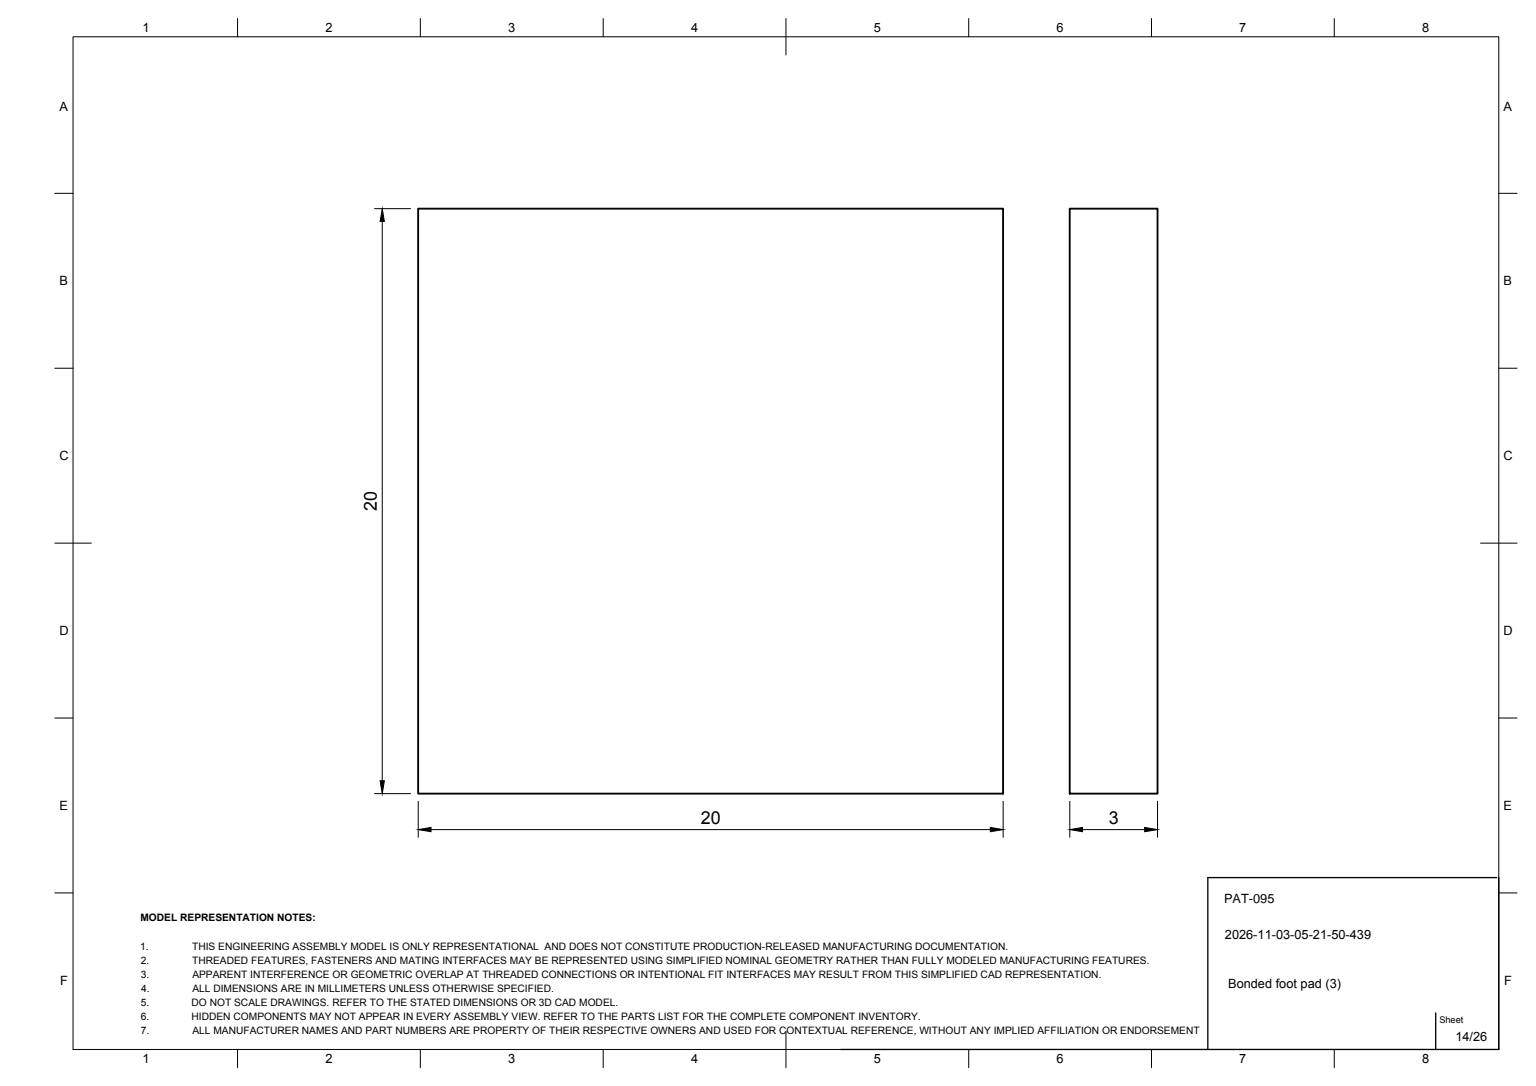
ISO-10303-21;
HEADER;
/* Generated by software containing ST-Developer
 * from STEP Tools, Inc. (www.steptools.com) 
 */

FILE_DESCRIPTION(
/* description */ ('Single-Axis Profile-Rail Linear Slide'),
/* implementation_level */ '2;1');

FILE_NAME(
/* name */ 'Bonded foot pad (3).step',
/* time_stamp */ '2026-10-27T10:47:43-07:00',
/* author */ (''),
/* organization */ (''),
/* preprocessor_version */ 'ST-DEVELOPER v20.2',
/* originating_system */ 'Autodesk Translation Framework v15.17.0.0',
/* authorisation */ '');

FILE_SCHEMA (('AUTOMOTIVE_DESIGN { 1 0 10303 214 3 1 1 }'));
ENDSEC;

DATA;
#10=MECHANICAL_DESIGN_GEOMETRIC_PRESENTATION_REPRESENTATION('',(#338),#14478);
#284=SHAPE_REPRESENTATION_RELATIONSHIP('SRR','None',#14614,#311);
#311=ADVANCED_BREP_SHAPE_REPRESENTATION('',(#365),#14458);
#338=STYLED_ITEM('',(#14824),#365);
#365=MANIFOLD_SOLID_BREP('Body1',#8598);
#642=PLANE('',#9177);
#643=PLANE('',#9178);
#644=PLANE('',#9179);
#645=PLANE('',#9180);
#646=PLANE('',#9181);
#647=PLANE('',#9182);
#1038=FACE_OUTER_BOUND('',#1537,.T.);
#1039=FACE_OUTER_BOUND('',#1538,.T.);
#1040=FACE_OUTER_BOUND('',#1539,.T.);
#1041=FACE_OUTER_BOUND('',#1540,.T.);
#1042=FACE_OUTER_BOUND('',#1541,.T.);
#1043=FACE_OUTER_BOUND('',#1542,.T.);
#1537=EDGE_LOOP('',(#6869,#6870,#6871,#6872));
#1538=EDGE_LOOP('',(#6873,#6874,#6875,#6876));
#1539=EDGE_LOOP('',(#6877,#6878,#6879,#6880));
#1540=EDGE_LOOP('',(#6881,#6882,#6883,#6884));
#1541=EDGE_LOOP('',(#6885,#6886,#6887,#6888));
#1542=EDGE_LOOP('',(#6889,#6890,#6891,#6892));
#2320=LINE('',#13089,#3291);
#2321=LINE('',#13091,#3292);
#2322=LINE('',#13093,#3293);
#2323=LINE('',#13094,#3294);
#2324=LINE('',#13097,#3295);
#2325=LINE('',#13099,#3296);
#2326=LINE('',#13100,#3297);
#2327=LINE('',#13103,#3298);
#2328=LINE('',#13105,#3299);
#2329=LINE('',#13106,#3300);
#2330=LINE('',#13108,#3301);
#2331=LINE('',#13109,#3302);
#3291=VECTOR('',#10619,1.);
#3292=VECTOR('',#10620,1.);
#3293=VECTOR('',#10621,1.);
#3294=VECTOR('',#10622,1.);
#3295=VECTOR('',#10625,1.);
#3296=VECTOR('',#10626,1.);
#3297=VECTOR('',#10627,1.);
#3298=VECTOR('',#10630,1.);
#3299=VECTOR('',#10631,1.);
#3300=VECTOR('',#10632,1.);
#3301=VECTOR('',#10635,1.);
#3302=VECTOR('',#10636,1.);
#4290=VERTEX_POINT('',#13087);
#4291=VERTEX_POINT('',#13088);
#4292=VERTEX_POINT('',#13090);
#4293=VERTEX_POINT('',#13092);
#4294=VERTEX_POINT('',#13096);
#4295=VERTEX_POINT('',#13098);
#4296=VERTEX_POINT('',#13102);
#4297=VERTEX_POINT('',#13104);
#5212=EDGE_CURVE('',#4290,#4291,#2320,.T.);
#5213=EDGE_CURVE('',#4291,#4292,#2321,.T.);
#5214=EDGE_CURVE('',#4293,#4292,#2322,.T.);
#5215=EDGE_CURVE('',#4290,#4293,#2323,.T.);
#5216=EDGE_CURVE('',#4294,#4290,#2324,.T.);
#5217=EDGE_CURVE('',#4295,#4293,#2325,.T.);
#5218=EDGE_CURVE('',#4294,#4295,#2326,.T.);
#5219=EDGE_CURVE('',#4296,#4294,#2327,.T.);
#5220=EDGE_CURVE('',#4297,#4295,#2328,.T.);
#5221=EDGE_CURVE('',#4296,#4297,#2329,.T.);
#5222=EDGE_CURVE('',#4291,#4296,#2330,.T.);
#5223=EDGE_CURVE('',#4292,#4297,#2331,.T.);
#6869=ORIENTED_EDGE('',*,*,#5212,.T.);
#6870=ORIENTED_EDGE('',*,*,#5213,.T.);
#6871=ORIENTED_EDGE('',*,*,#5214,.F.);
#6872=ORIENTED_EDGE('',*,*,#5215,.F.);
#6873=ORIENTED_EDGE('',*,*,#5216,.T.);
#6874=ORIENTED_EDGE('',*,*,#5215,.T.);
#6875=ORIENTED_EDGE('',*,*,#5217,.F.);
#6876=ORIENTED_EDGE('',*,*,#5218,.F.);
#6877=ORIENTED_EDGE('',*,*,#5219,.T.);
#6878=ORIENTED_EDGE('',*,*,#5218,.T.);
#6879=ORIENTED_EDGE('',*,*,#5220,.F.);
#6880=ORIENTED_EDGE('',*,*,#5221,.F.);
#6881=ORIENTED_EDGE('',*,*,#5222,.T.);
#6882=ORIENTED_EDGE('',*,*,#5221,.T.);
#6883=ORIENTED_EDGE('',*,*,#5223,.F.);
#6884=ORIENTED_EDGE('',*,*,#5213,.F.);
#6885=ORIENTED_EDGE('',*,*,#5223,.T.);
#6886=ORIENTED_EDGE('',*,*,#5220,.T.);
#6887=ORIENTED_EDGE('',*,*,#5217,.T.);
#6888=ORIENTED_EDGE('',*,*,#5214,.T.);
#6889=ORIENTED_EDGE('',*,*,#5222,.F.);
#6890=ORIENTED_EDGE('',*,*,#5212,.F.);
#6891=ORIENTED_EDGE('',*,*,#5216,.F.);
#6892=ORIENTED_EDGE('',*,*,#5219,.F.);
#8332=ADVANCED_FACE('',(#1038),#642,.T.);
#8333=ADVANCED_FACE('',(#1039),#643,.T.);
#8334=ADVANCED_FACE('',(#1040),#644,.T.);
#8335=ADVANCED_FACE('',(#1041),#645,.T.);
#8336=ADVANCED_FACE('',(#1042),#646,.T.);
#8337=ADVANCED_FACE('',(#1043),#647,.F.);
#8598=CLOSED_SHELL('',(#8332,#8333,#8334,#8335,#8336,#8337));
#9176=AXIS2_PLACEMENT_3D('',#13085,#10615,#10616);
#9177=AXIS2_PLACEMENT_3D('',#13086,#10617,#10618);
#9178=AXIS2_PLACEMENT_3D('',#13095,#10623,#10624);
#9179=AXIS2_PLACEMENT_3D('',#13101,#10628,#10629);
#9180=AXIS2_PLACEMENT_3D('',#13107,#10633,#10634);
#9181=AXIS2_PLACEMENT_3D('',#13110,#10637,#10638);
#9182=AXIS2_PLACEMENT_3D('',#13111,#10639,#10640);
#10615=DIRECTION('axis',(0.,0.,1.));
#10616=DIRECTION('refdir',(1.,0.,0.));
#10617=DIRECTION('center_axis',(0.,1.,0.));
#10618=DIRECTION('ref_axis',(-1.,0.,0.));
#10619=DIRECTION('',(-1.,0.,0.));
#10620=DIRECTION('',(0.,0.,1.));
#10621=DIRECTION('',(-1.,0.,0.));
#10622=DIRECTION('',(0.,0.,1.));
#10623=DIRECTION('center_axis',(1.,0.,0.));
#10624=DIRECTION('ref_axis',(0.,1.,0.));
#10625=DIRECTION('',(0.,1.,0.));
#10626=DIRECTION('',(0.,1.,0.));
#10627=DIRECTION('',(0.,0.,1.));
#10628=DIRECTION('center_axis',(0.,-1.,0.));
#10629=DIRECTION('ref_axis',(1.,0.,0.));
#10630=DIRECTION('',(1.,0.,0.));
#10631=DIRECTION('',(1.,0.,0.));
#10632=DIRECTION('',(0.,0.,1.));
#10633=DIRECTION('center_axis',(-1.,0.,0.));
#10634=DIRECTION('ref_axis',(0.,-1.,0.));
#10635=DIRECTION('',(0.,-1.,0.));
#10636=DIRECTION('',(0.,-1.,0.));
#10637=DIRECTION('center_axis',(0.,0.,1.));
#10638=DIRECTION('ref_axis',(1.,0.,0.));
#10639=DIRECTION('center_axis',(0.,0.,1.));
#10640=DIRECTION('ref_axis',(1.,0.,0.));
#13085=CARTESIAN_POINT('',(0.,0.,0.));
#13086=CARTESIAN_POINT('Origin',(20.,4.5,-0.3));
#13087=CARTESIAN_POINT('',(20.,4.5,-0.3));
#13088=CARTESIAN_POINT('',(18.,4.5,-0.3));
#13089=CARTESIAN_POINT('',(20.,4.5,-0.3));
#13090=CARTESIAN_POINT('',(18.,4.5,0.));
#13091=CARTESIAN_POINT('',(18.,4.5,-0.3));
#13092=CARTESIAN_POINT('',(20.,4.5,0.));
#13093=CARTESIAN_POINT('',(20.,4.5,0.));
#13094=CARTESIAN_POINT('',(20.,4.5,-0.3));
#13095=CARTESIAN_POINT('Origin',(20.,2.5,-0.3));
#13096=CARTESIAN_POINT('',(20.,2.5,-0.3));
#13097=CARTESIAN_POINT('',(20.,2.5,-0.3));
#13098=CARTESIAN_POINT('',(20.,2.5,0.));
#13099=CARTESIAN_POINT('',(20.,2.5,0.));
#13100=CARTESIAN_POINT('',(20.,2.5,-0.3));
#13101=CARTESIAN_POINT('Origin',(18.,2.5,-0.3));
#13102=CARTESIAN_POINT('',(18.,2.5,-0.3));
#13103=CARTESIAN_POINT('',(18.,2.5,-0.3));
#13104=CARTESIAN_POINT('',(18.,2.5,0.));
#13105=CARTESIAN_POINT('',(18.,2.5,0.));
#13106=CARTESIAN_POINT('',(18.,2.5,-0.3));
#13107=CARTESIAN_POINT('Origin',(18.,4.5,-0.3));
#13108=CARTESIAN_POINT('',(18.,4.5,-0.3));
#13109=CARTESIAN_POINT('',(18.,4.5,0.));
#13110=CARTESIAN_POINT('Origin',(19.,3.5,0.));
#13111=CARTESIAN_POINT('Origin',(19.,3.5,-0.3));
#14426=UNCERTAINTY_MEASURE_WITH_UNIT(LENGTH_MEASURE(0.001),#14479,
'DISTANCE_ACCURACY_VALUE',
'Maximum model space distance between geometric entities at asserted c
onnectivities');
#14446=UNCERTAINTY_MEASURE_WITH_UNIT(LENGTH_MEASURE(0.001),#14479,
'DISTANCE_ACCURACY_VALUE',
'Maximum model space distance between geometric entities at asserted c
onnectivities');
#14458=(
GEOMETRIC_REPRESENTATION_CONTEXT(3)
GLOBAL_UNCERTAINTY_ASSIGNED_CONTEXT((#14426))
GLOBAL_UNIT_ASSIGNED_CONTEXT((#14479,#14481,#14482))
REPRESENTATION_CONTEXT('','3D')
);
#14478=(
GEOMETRIC_REPRESENTATION_CONTEXT(3)
GLOBAL_UNCERTAINTY_ASSIGNED_CONTEXT((#14446))
GLOBAL_UNIT_ASSIGNED_CONTEXT((#14479,#14481,#14482))
REPRESENTATION_CONTEXT('','3D')
);
#14479=(
LENGTH_UNIT()
NAMED_UNIT(*)
SI_UNIT(.CENTI.,.METRE.)
);
#14481=(
NAMED_UNIT(*)
PLANE_ANGLE_UNIT()
SI_UNIT($,.RADIAN.)
);
#14482=(
NAMED_UNIT(*)
SI_UNIT($,.STERADIAN.)
SOLID_ANGLE_UNIT()
);
#14494=SHAPE_DEFINITION_REPRESENTATION(#14525,#14614);
#14525=PRODUCT_DEFINITION_SHAPE('',$,#14646);
#14614=SHAPE_REPRESENTATION('',(#9176),#14458);
#14634=PRODUCT_DEFINITION_CONTEXT('part definition',#14729,'design');
#14646=PRODUCT_DEFINITION('Bonded foot pad (3)','Bonded foot pad (3)',#14677,
#14634);
#14677=PRODUCT_DEFINITION_FORMATION('',$,#14742);
#14729=APPLICATION_CONTEXT(
'Core Data for Automotive Mechanical Design Process');
#14730=PRODUCT_CONTEXT('part definition',#14729,'mechanical');
#14742=PRODUCT('Bonded foot pad (3)','Bonded foot pad (3)',
'Bonded foot pad (3)',(#14730));
#14818=COLOUR_RGB('Sky Blue',0.24,0.69,0.87);
#14819=FILL_AREA_STYLE_COLOUR('',#14818);
#14820=FILL_AREA_STYLE('',(#14819));
#14821=SURFACE_STYLE_FILL_AREA(#14820);
#14822=SURFACE_SIDE_STYLE('',(#14821));
#14823=SURFACE_STYLE_USAGE(.BOTH.,#14822);
#14824=PRESENTATION_STYLE_ASSIGNMENT((#14823));
ENDSEC;
END-ISO-10303-21;
